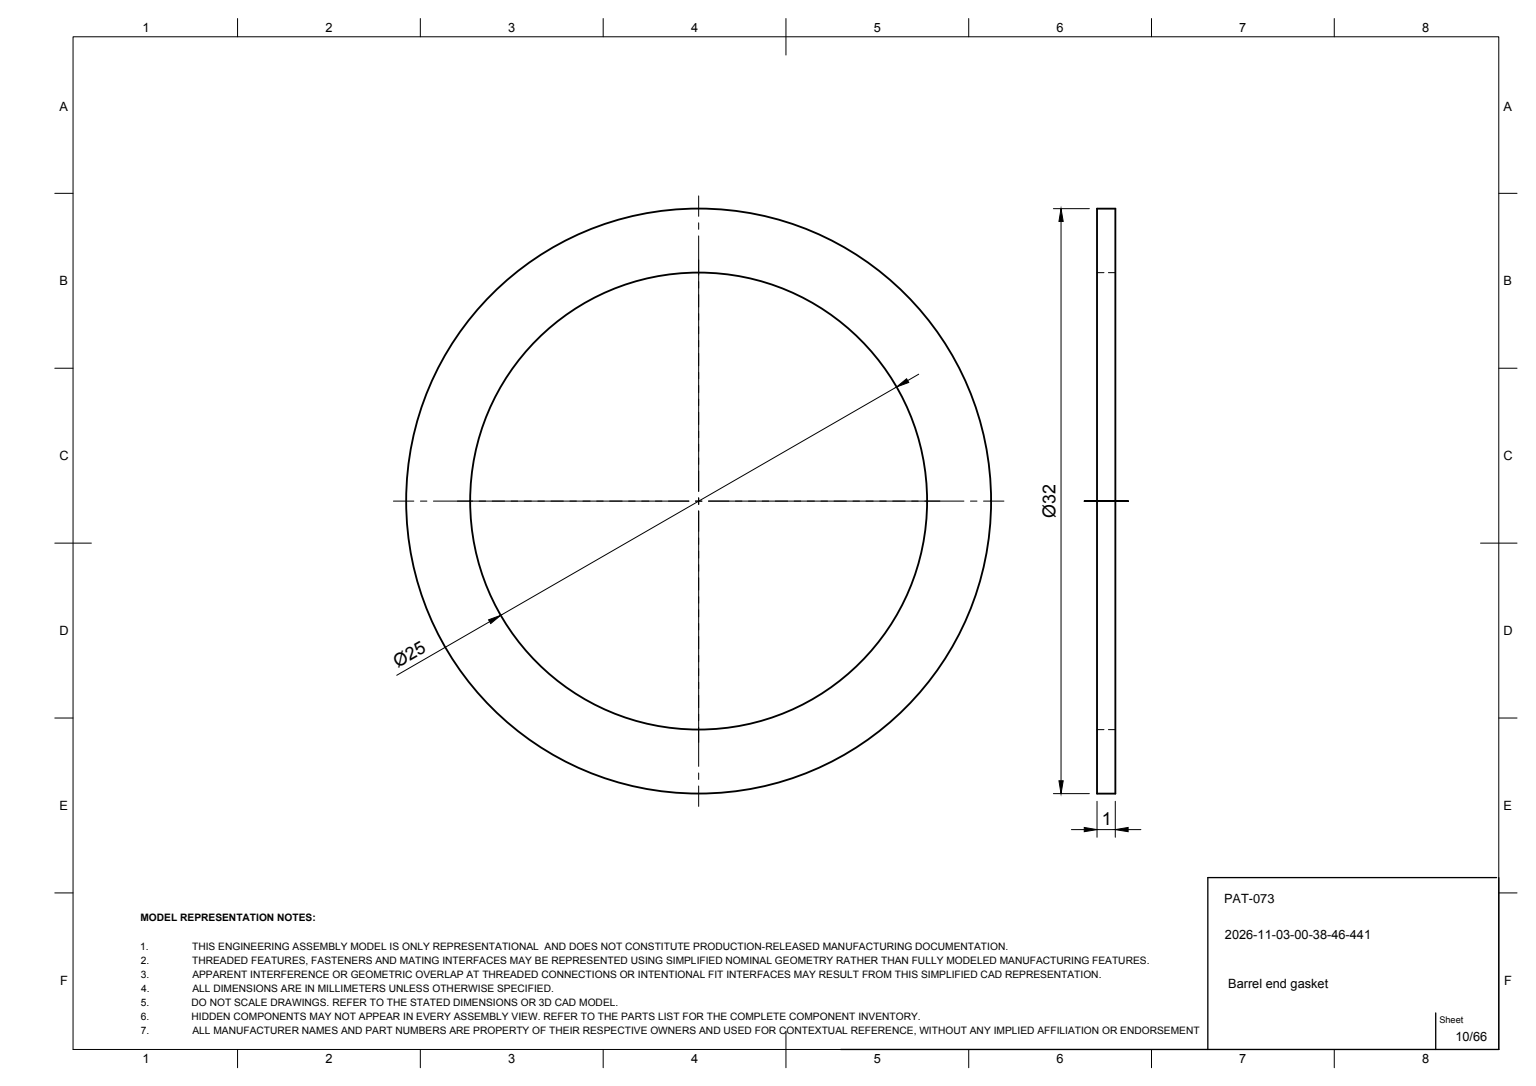
ISO-10303-21;
HEADER;
/* Generated by software containing ST-Developer
 * from STEP Tools, Inc. (www.steptools.com) 
 */

FILE_DESCRIPTION(
/* description */ ('Manual piston pump'),
/* implementation_level */ '2;1');

FILE_NAME(
/* name */ 'Barrel end gasket.step',
/* time_stamp */ '2026-11-02T16:54:23-08:00',
/* author */ (''),
/* organization */ (''),
/* preprocessor_version */ 'ST-DEVELOPER v20.2',
/* originating_system */ 'Autodesk Translation Framework v15.17.0.0',
/* authorisation */ '');

FILE_SCHEMA (('AUTOMOTIVE_DESIGN { 1 0 10303 214 3 1 1 }'));
ENDSEC;

DATA;
#10=MECHANICAL_DESIGN_GEOMETRIC_PRESENTATION_REPRESENTATION('',(#693),#19043);
#567=SHAPE_REPRESENTATION_RELATIONSHIP('SRR','None',#19313,#630);
#630=ADVANCED_BREP_SHAPE_REPRESENTATION('',(#765),#18980);
#693=STYLED_ITEM('',(#19661),#765);
#765=MANIFOLD_SOLID_BREP('Body1',#9477);
#876=FACE_BOUND('',#2003,.T.);
#877=FACE_BOUND('',#2005,.T.);
#1130=CYLINDRICAL_SURFACE('',#10415,1.25);
#1131=CYLINDRICAL_SURFACE('',#10418,1.6);
#1376=FACE_OUTER_BOUND('',#2000,.T.);
#1377=FACE_OUTER_BOUND('',#2001,.T.);
#1378=FACE_OUTER_BOUND('',#2002,.T.);
#1379=FACE_OUTER_BOUND('',#2004,.T.);
#2000=EDGE_LOOP('',(#6659,#6660,#6661,#6662));
#2001=EDGE_LOOP('',(#6663,#6664,#6665,#6666));
#2002=EDGE_LOOP('',(#6667));
#2003=EDGE_LOOP('',(#6668));
#2004=EDGE_LOOP('',(#6669));
#2005=EDGE_LOOP('',(#6670));
#2743=CIRCLE('',#10416,1.25);
#2744=CIRCLE('',#10417,1.25);
#2745=CIRCLE('',#10419,1.6);
#2746=CIRCLE('',#10420,1.6);
#3257=LINE('',#15071,#3861);
#3258=LINE('',#15077,#3862);
#3861=VECTOR('',#11953,1.25);
#3862=VECTOR('',#11960,1.6);
#4483=VERTEX_POINT('',#15068);
#4484=VERTEX_POINT('',#15070);
#4485=VERTEX_POINT('',#15074);
#4486=VERTEX_POINT('',#15076);
#5316=EDGE_CURVE('',#4483,#4483,#2743,.T.);
#5317=EDGE_CURVE('',#4483,#4484,#3257,.T.);
#5318=EDGE_CURVE('',#4484,#4484,#2744,.T.);
#5319=EDGE_CURVE('',#4485,#4485,#2745,.T.);
#5320=EDGE_CURVE('',#4485,#4486,#3258,.T.);
#5321=EDGE_CURVE('',#4486,#4486,#2746,.T.);
#6659=ORIENTED_EDGE('',*,*,#5316,.F.);
#6660=ORIENTED_EDGE('',*,*,#5317,.T.);
#6661=ORIENTED_EDGE('',*,*,#5318,.T.);
#6662=ORIENTED_EDGE('',*,*,#5317,.F.);
#6663=ORIENTED_EDGE('',*,*,#5319,.F.);
#6664=ORIENTED_EDGE('',*,*,#5320,.T.);
#6665=ORIENTED_EDGE('',*,*,#5321,.T.);
#6666=ORIENTED_EDGE('',*,*,#5320,.F.);
#6667=ORIENTED_EDGE('',*,*,#5319,.T.);
#6668=ORIENTED_EDGE('',*,*,#5316,.T.);
#6669=ORIENTED_EDGE('',*,*,#5321,.F.);
#6670=ORIENTED_EDGE('',*,*,#5318,.F.);
#8618=PLANE('',#10421);
#8619=PLANE('',#10422);
#8981=ADVANCED_FACE('',(#1376),#1130,.F.);
#8982=ADVANCED_FACE('',(#1377),#1131,.T.);
#8983=ADVANCED_FACE('',(#1378,#876),#8618,.T.);
#8984=ADVANCED_FACE('',(#1379,#877),#8619,.F.);
#9477=CLOSED_SHELL('',(#8981,#8982,#8983,#8984));
#10414=AXIS2_PLACEMENT_3D('',#15066,#11947,#11948);
#10415=AXIS2_PLACEMENT_3D('',#15067,#11949,#11950);
#10416=AXIS2_PLACEMENT_3D('',#15069,#11951,#11952);
#10417=AXIS2_PLACEMENT_3D('',#15072,#11954,#11955);
#10418=AXIS2_PLACEMENT_3D('',#15073,#11956,#11957);
#10419=AXIS2_PLACEMENT_3D('',#15075,#11958,#11959);
#10420=AXIS2_PLACEMENT_3D('',#15078,#11961,#11962);
#10421=AXIS2_PLACEMENT_3D('',#15079,#11963,#11964);
#10422=AXIS2_PLACEMENT_3D('',#15080,#11965,#11966);
#11947=DIRECTION('axis',(0.,0.,1.));
#11948=DIRECTION('refdir',(1.,0.,0.));
#11949=DIRECTION('center_axis',(0.,1.,0.));
#11950=DIRECTION('ref_axis',(1.,0.,0.));
#11951=DIRECTION('center_axis',(0.,-1.,0.));
#11952=DIRECTION('ref_axis',(1.,0.,0.));
#11953=DIRECTION('',(0.,-1.,0.));
#11954=DIRECTION('center_axis',(0.,-1.,0.));
#11955=DIRECTION('ref_axis',(1.,0.,0.));
#11956=DIRECTION('center_axis',(0.,1.,0.));
#11957=DIRECTION('ref_axis',(1.,0.,0.));
#11958=DIRECTION('center_axis',(0.,1.,0.));
#11959=DIRECTION('ref_axis',(1.,0.,0.));
#11960=DIRECTION('',(0.,-1.,0.));
#11961=DIRECTION('center_axis',(0.,1.,0.));
#11962=DIRECTION('ref_axis',(1.,0.,0.));
#11963=DIRECTION('center_axis',(0.,1.,0.));
#11964=DIRECTION('ref_axis',(1.,0.,0.));
#11965=DIRECTION('center_axis',(0.,1.,0.));
#11966=DIRECTION('ref_axis',(1.,0.,0.));
#15066=CARTESIAN_POINT('',(0.,0.,0.));
#15067=CARTESIAN_POINT('Origin',(0.,1.7,4.5));
#15068=CARTESIAN_POINT('',(-1.25,1.8,4.5));
#15069=CARTESIAN_POINT('Origin',(0.,1.8,4.5));
#15070=CARTESIAN_POINT('',(-1.25,1.7,4.5));
#15071=CARTESIAN_POINT('',(-1.25,1.7,4.5));
#15072=CARTESIAN_POINT('Origin',(0.,1.7,4.5));
#15073=CARTESIAN_POINT('Origin',(0.,1.7,4.5));
#15074=CARTESIAN_POINT('',(-1.6,1.8,4.5));
#15075=CARTESIAN_POINT('Origin',(0.,1.8,4.5));
#15076=CARTESIAN_POINT('',(-1.6,1.7,4.5));
#15077=CARTESIAN_POINT('',(-1.6,1.7,4.5));
#15078=CARTESIAN_POINT('Origin',(0.,1.7,4.5));
#15079=CARTESIAN_POINT('Origin',(0.,1.8,4.5));
#15080=CARTESIAN_POINT('Origin',(0.,1.7,4.5));
#18909=UNCERTAINTY_MEASURE_WITH_UNIT(LENGTH_MEASURE(0.001),#19044,
'DISTANCE_ACCURACY_VALUE',
'Maximum model space distance between geometric entities at asserted c
onnectivities');
#18972=UNCERTAINTY_MEASURE_WITH_UNIT(LENGTH_MEASURE(0.001),#19044,
'DISTANCE_ACCURACY_VALUE',
'Maximum model space distance between geometric entities at asserted c
onnectivities');
#18980=(
GEOMETRIC_REPRESENTATION_CONTEXT(3)
GLOBAL_UNCERTAINTY_ASSIGNED_CONTEXT((#18909))
GLOBAL_UNIT_ASSIGNED_CONTEXT((#19044,#19046,#19047))
REPRESENTATION_CONTEXT('','3D')
);
#19043=(
GEOMETRIC_REPRESENTATION_CONTEXT(3)
GLOBAL_UNCERTAINTY_ASSIGNED_CONTEXT((#18972))
GLOBAL_UNIT_ASSIGNED_CONTEXT((#19044,#19046,#19047))
REPRESENTATION_CONTEXT('','3D')
);
#19044=(
LENGTH_UNIT()
NAMED_UNIT(*)
SI_UNIT(.CENTI.,.METRE.)
);
#19046=(
NAMED_UNIT(*)
PLANE_ANGLE_UNIT()
SI_UNIT($,.RADIAN.)
);
#19047=(
NAMED_UNIT(*)
SI_UNIT($,.STERADIAN.)
SOLID_ANGLE_UNIT()
);
#19055=SHAPE_DEFINITION_REPRESENTATION(#19125,#19313);
#19125=PRODUCT_DEFINITION_SHAPE('',$,#19384);
#19313=SHAPE_REPRESENTATION('',(#10414),#18980);
#19376=PRODUCT_DEFINITION_CONTEXT('part definition',#19588,'design');
#19384=PRODUCT_DEFINITION('2026-11-03-00-38-46-441','Barrel end gasket',
#19454,#19376);
#19454=PRODUCT_DEFINITION_FORMATION('',$,#19597);
#19588=APPLICATION_CONTEXT(
'Core Data for Automotive Mechanical Design Process');
#19589=PRODUCT_CONTEXT('part definition',#19588,'mechanical');
#19597=PRODUCT('2026-11-03-00-38-46-441','Barrel end gasket',
'Barrel end gasket',(#19589));
#19661=PRESENTATION_STYLE_ASSIGNMENT((#19667));
#19667=SURFACE_STYLE_USAGE(.BOTH.,#19673);
#19673=SURFACE_SIDE_STYLE('',(#19679));
#19679=SURFACE_STYLE_FILL_AREA(#19685);
#19685=FILL_AREA_STYLE('CAD Library Painted - Engineering blue',(#19691));
#19691=FILL_AREA_STYLE_COLOUR('CAD Library Painted - Engineering blue',
#19697);
#19697=COLOUR_RGB('CAD Library Painted - Engineering blue',0.12156862745098,
0.356862745098039,0.6);
ENDSEC;
END-ISO-10303-21;
